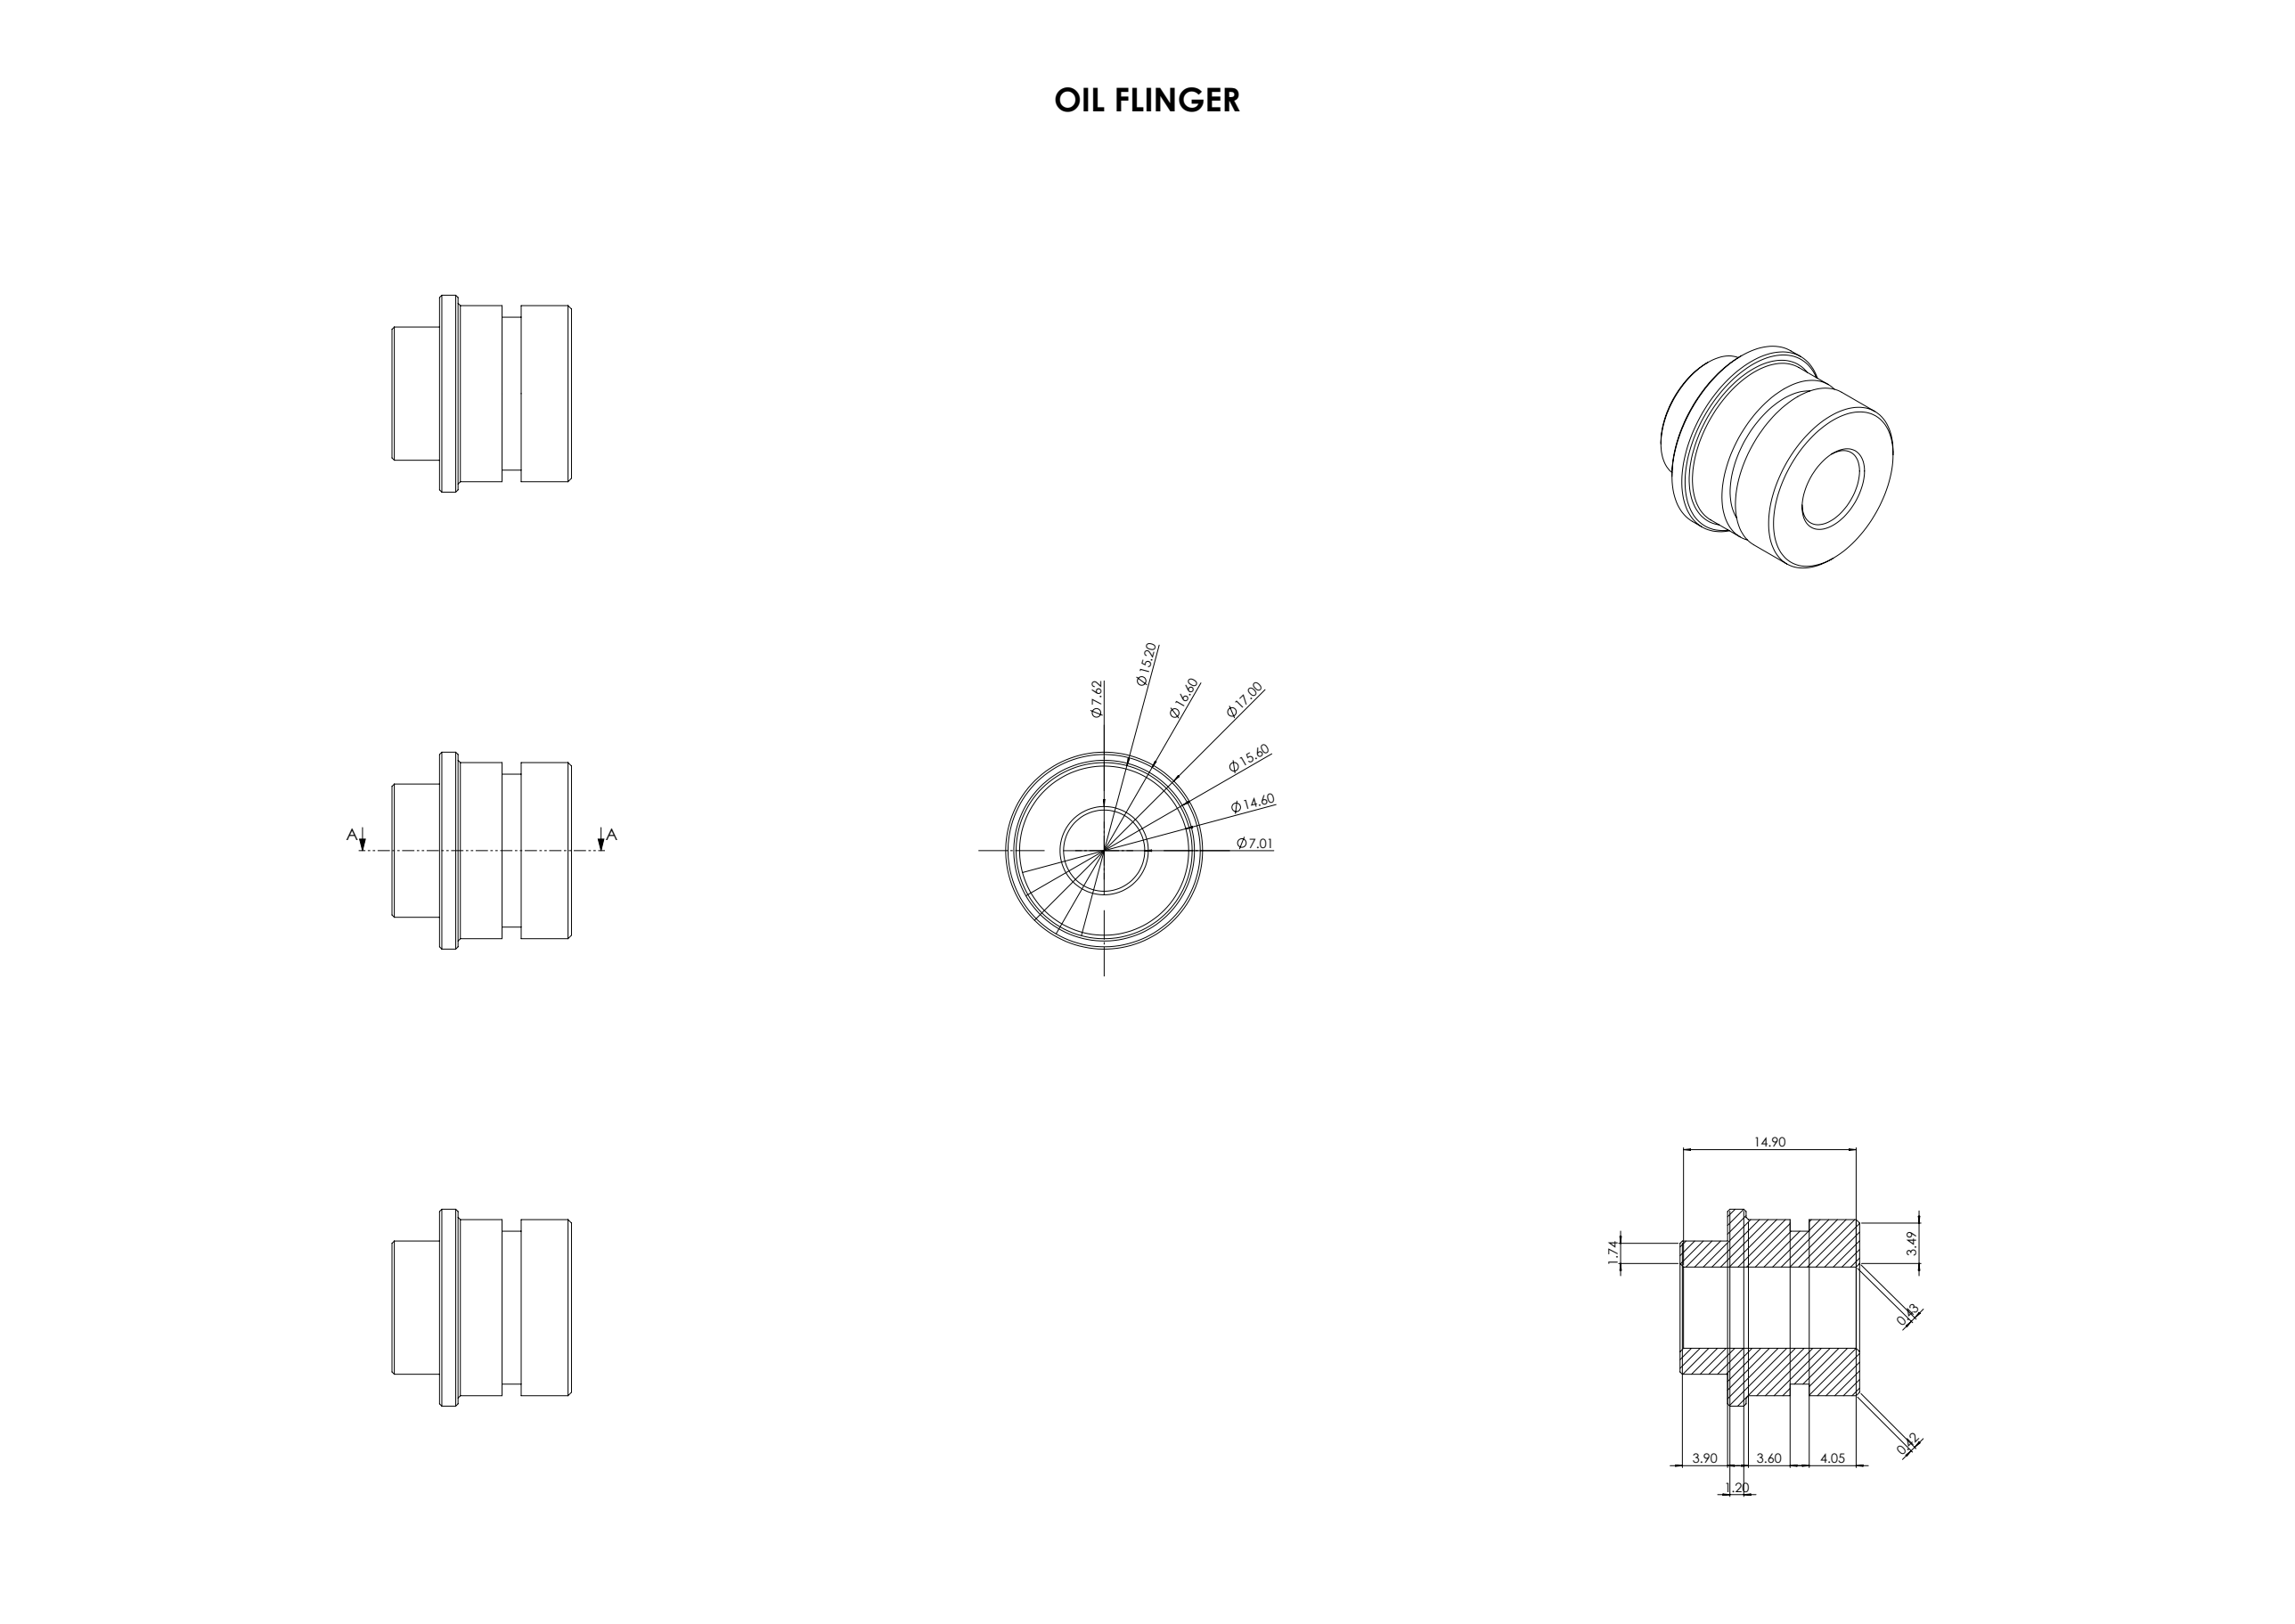
ISO-10303-21;
HEADER;
/* Generated by software containing ST-Developer
 * from STEP Tools, Inc. (www.steptools.com) 
 */

FILE_DESCRIPTION(
/* description */ (''),
/* implementation_level */ '2;1');

FILE_NAME(
/* name */ '07_Oil_Flinger.step',
/* time_stamp */ '2026-10-25T01:10:36-07:00',
/* author */ (''),
/* organization */ (''),
/* preprocessor_version */ 'ST-DEVELOPER v20.2',
/* originating_system */ 'Autodesk Translation Framework v15.15.0.0',
/* authorisation */ '');

FILE_SCHEMA (('AUTOMOTIVE_DESIGN { 1 0 10303 214 3 1 1 }'));
ENDSEC;

DATA;
#10=MECHANICAL_DESIGN_GEOMETRIC_PRESENTATION_REPRESENTATION('',(#1299),#60365);
#71=SHAPE_REPRESENTATION_RELATIONSHIP('SRR','None',#60411,#81);
#81=ADVANCED_BREP_SHAPE_REPRESENTATION('',(#91),#60359);
#91=MANIFOLD_SOLID_BREP('Body1',#18301);
#229=FACE_BOUND('',#2864,.T.);
#230=FACE_BOUND('',#2866,.T.);
#231=FACE_BOUND('',#2871,.T.);
#232=FACE_BOUND('',#2872,.T.);
#233=FACE_BOUND('',#2873,.T.);
#234=FACE_BOUND('',#2874,.T.);
#235=FACE_BOUND('',#2875,.T.);
#236=FACE_BOUND('',#2876,.T.);
#237=FACE_BOUND('',#2877,.T.);
#238=FACE_BOUND('',#2882,.T.);
#239=FACE_BOUND('',#2887,.T.);
#240=FACE_BOUND('',#2892,.T.);
#592=PLANE('',#19167);
#593=PLANE('',#19171);
#594=PLANE('',#19175);
#595=PLANE('',#19179);
#596=PLANE('',#19183);
#597=PLANE('',#19187);
#598=PLANE('',#19191);
#599=PLANE('',#19193);
#600=PLANE('',#19202);
#601=PLANE('',#19210);
#602=PLANE('',#19217);
#603=PLANE('',#19225);
#915=CONICAL_SURFACE('',#19197,5.65,0.785398163397449);
#916=CONICAL_SURFACE('',#19204,8.4,0.785398163397446);
#917=CONICAL_SURFACE('',#19208,8.4,0.785398163397446);
#918=CONICAL_SURFACE('',#19212,7.7,0.785398163397448);
#919=CONICAL_SURFACE('',#19215,7.45,0.785398163397448);
#920=CONICAL_SURFACE('',#19219,3.6575,0.7936624380571);
#921=CONICAL_SURFACE('',#19223,3.6575,0.7936624380571);
#1299=STYLED_ITEM('',(#60520),#91);
#1854=FACE_OUTER_BOUND('',#2850,.T.);
#1855=FACE_OUTER_BOUND('',#2851,.T.);
#1856=FACE_OUTER_BOUND('',#2852,.T.);
#1857=FACE_OUTER_BOUND('',#2853,.T.);
#1858=FACE_OUTER_BOUND('',#2854,.T.);
#1859=FACE_OUTER_BOUND('',#2855,.T.);
#1860=FACE_OUTER_BOUND('',#2856,.T.);
#1861=FACE_OUTER_BOUND('',#2857,.T.);
#1862=FACE_OUTER_BOUND('',#2858,.T.);
#1863=FACE_OUTER_BOUND('',#2859,.T.);
#1864=FACE_OUTER_BOUND('',#2860,.T.);
#1865=FACE_OUTER_BOUND('',#2861,.T.);
#1866=FACE_OUTER_BOUND('',#2862,.T.);
#1867=FACE_OUTER_BOUND('',#2863,.T.);
#1868=FACE_OUTER_BOUND('',#2865,.T.);
#1869=FACE_OUTER_BOUND('',#2867,.T.);
#1870=FACE_OUTER_BOUND('',#2868,.T.);
#1871=FACE_OUTER_BOUND('',#2869,.T.);
#1872=FACE_OUTER_BOUND('',#2870,.T.);
#1873=FACE_OUTER_BOUND('',#2878,.T.);
#1874=FACE_OUTER_BOUND('',#2879,.T.);
#1875=FACE_OUTER_BOUND('',#2880,.T.);
#1876=FACE_OUTER_BOUND('',#2881,.T.);
#1877=FACE_OUTER_BOUND('',#2883,.T.);
#1878=FACE_OUTER_BOUND('',#2884,.T.);
#1879=FACE_OUTER_BOUND('',#2885,.T.);
#1880=FACE_OUTER_BOUND('',#2886,.T.);
#1881=FACE_OUTER_BOUND('',#2888,.T.);
#1882=FACE_OUTER_BOUND('',#2889,.T.);
#1883=FACE_OUTER_BOUND('',#2890,.T.);
#1884=FACE_OUTER_BOUND('',#2891,.T.);
#2850=EDGE_LOOP('',(#14883,#14884,#14885,#14886));
#2851=EDGE_LOOP('',(#14887));
#2852=EDGE_LOOP('',(#14888,#14889,#14890,#14891));
#2853=EDGE_LOOP('',(#14892));
#2854=EDGE_LOOP('',(#14893,#14894,#14895,#14896));
#2855=EDGE_LOOP('',(#14897));
#2856=EDGE_LOOP('',(#14898,#14899,#14900,#14901));
#2857=EDGE_LOOP('',(#14902));
#2858=EDGE_LOOP('',(#14903,#14904,#14905,#14906));
#2859=EDGE_LOOP('',(#14907));
#2860=EDGE_LOOP('',(#14908,#14909,#14910,#14911));
#2861=EDGE_LOOP('',(#14912));
#2862=EDGE_LOOP('',(#14913,#14914,#14915,#14916));
#2863=EDGE_LOOP('',(#14917));
#2864=EDGE_LOOP('',(#14918));
#2865=EDGE_LOOP('',(#14919));
#2866=EDGE_LOOP('',(#14920));
#2867=EDGE_LOOP('',(#14921,#14922,#14923,#14924));
#2868=EDGE_LOOP('',(#14925,#14926,#14927,#14928));
#2869=EDGE_LOOP('',(#14929,#14930,#14931,#14932));
#2870=EDGE_LOOP('',(#14933));
#2871=EDGE_LOOP('',(#14934));
#2872=EDGE_LOOP('',(#14935));
#2873=EDGE_LOOP('',(#14936));
#2874=EDGE_LOOP('',(#14937));
#2875=EDGE_LOOP('',(#14938));
#2876=EDGE_LOOP('',(#14939));
#2877=EDGE_LOOP('',(#14940));
#2878=EDGE_LOOP('',(#14941,#14942,#14943,#14944));
#2879=EDGE_LOOP('',(#14945,#14946,#14947,#14948));
#2880=EDGE_LOOP('',(#14949,#14950,#14951,#14952));
#2881=EDGE_LOOP('',(#14953));
#2882=EDGE_LOOP('',(#14954));
#2883=EDGE_LOOP('',(#14955,#14956,#14957,#14958));
#2884=EDGE_LOOP('',(#14959,#14960,#14961,#14962));
#2885=EDGE_LOOP('',(#14963,#14964,#14965,#14966));
#2886=EDGE_LOOP('',(#14967));
#2887=EDGE_LOOP('',(#14968));
#2888=EDGE_LOOP('',(#14969,#14970,#14971,#14972));
#2889=EDGE_LOOP('',(#14973,#14974,#14975,#14976));
#2890=EDGE_LOOP('',(#14977,#14978,#14979,#14980));
#2891=EDGE_LOOP('',(#14981));
#2892=EDGE_LOOP('',(#14982));
#3537=CIRCLE('',#19165,0.600000000000001);
#3538=CIRCLE('',#19166,0.600000000000001);
#3539=CIRCLE('',#19169,0.6);
#3540=CIRCLE('',#19170,0.6);
#3541=CIRCLE('',#19173,0.600000000000001);
#3542=CIRCLE('',#19174,0.600000000000001);
#3543=CIRCLE('',#19177,0.600000000000001);
#3544=CIRCLE('',#19178,0.600000000000001);
#3545=CIRCLE('',#19181,0.6);
#3546=CIRCLE('',#19182,0.6);
#3547=CIRCLE('',#19185,0.600000000000001);
#3548=CIRCLE('',#19186,0.600000000000001);
#3549=CIRCLE('',#19189,6.6);
#3550=CIRCLE('',#19190,6.6);
#3551=CIRCLE('',#19192,7.6);
#3552=CIRCLE('',#19194,7.6);
#3553=CIRCLE('',#19196,7.6);
#3554=CIRCLE('',#19198,5.75);
#3555=CIRCLE('',#19199,5.55);
#3556=CIRCLE('',#19201,5.75);
#3557=CIRCLE('',#19203,8.3);
#3558=CIRCLE('',#19205,8.5);
#3559=CIRCLE('',#19207,8.5);
#3560=CIRCLE('',#19209,8.3);
#3561=CIRCLE('',#19211,7.8);
#3562=CIRCLE('',#19213,7.6);
#3563=CIRCLE('',#19216,7.3);
#3564=CIRCLE('',#19218,3.81);
#3565=CIRCLE('',#19220,3.505);
#3566=CIRCLE('',#19222,3.505);
#3567=CIRCLE('',#19224,3.81);
#5321=LINE('',#44964,#6733);
#5322=LINE('',#44971,#6734);
#5323=LINE('',#44978,#6735);
#5324=LINE('',#44985,#6736);
#5325=LINE('',#44992,#6737);
#5326=LINE('',#44999,#6738);
#5327=LINE('',#45006,#6739);
#5328=LINE('',#45017,#6740);
#5329=LINE('',#45022,#6741);
#5330=LINE('',#45027,#6742);
#5331=LINE('',#45034,#6743);
#5332=LINE('',#45038,#6744);
#5333=LINE('',#45042,#6745);
#5334=LINE('',#45049,#6746);
#5335=LINE('',#45051,#6747);
#5336=LINE('',#45055,#6748);
#5337=LINE('',#45061,#6749);
#5338=LINE('',#45065,#6750);
#5339=LINE('',#45069,#6751);
#6733=VECTOR('',#21995,0.600000000000001);
#6734=VECTOR('',#22004,0.6);
#6735=VECTOR('',#22013,0.600000000000001);
#6736=VECTOR('',#22022,0.600000000000001);
#6737=VECTOR('',#22031,0.6);
#6738=VECTOR('',#22040,0.600000000000001);
#6739=VECTOR('',#22049,6.6);
#6740=VECTOR('',#22064,7.6);
#6741=VECTOR('',#22069,5.65);
#6742=VECTOR('',#22076,5.75);
#6743=VECTOR('',#22085,8.4);
#6744=VECTOR('',#22090,8.5);
#6745=VECTOR('',#22095,8.4);
#6746=VECTOR('',#22104,7.7);
#6747=VECTOR('',#22107,7.6);
#6748=VECTOR('',#22112,7.45);
#6749=VECTOR('',#22119,3.6575);
#6750=VECTOR('',#22124,3.505);
#6751=VECTOR('',#22129,3.6575);
#8337=VERTEX_POINT('',#44961);
#8338=VERTEX_POINT('',#44963);
#8339=VERTEX_POINT('',#44968);
#8340=VERTEX_POINT('',#44970);
#8341=VERTEX_POINT('',#44975);
#8342=VERTEX_POINT('',#44977);
#8343=VERTEX_POINT('',#44982);
#8344=VERTEX_POINT('',#44984);
#8345=VERTEX_POINT('',#44989);
#8346=VERTEX_POINT('',#44991);
#8347=VERTEX_POINT('',#44996);
#8348=VERTEX_POINT('',#44998);
#8349=VERTEX_POINT('',#45003);
#8350=VERTEX_POINT('',#45005);
#8351=VERTEX_POINT('',#45009);
#8352=VERTEX_POINT('',#45012);
#8353=VERTEX_POINT('',#45015);
#8354=VERTEX_POINT('',#45019);
#8355=VERTEX_POINT('',#45021);
#8356=VERTEX_POINT('',#45025);
#8357=VERTEX_POINT('',#45029);
#8358=VERTEX_POINT('',#45032);
#8359=VERTEX_POINT('',#45036);
#8360=VERTEX_POINT('',#45040);
#8361=VERTEX_POINT('',#45044);
#8362=VERTEX_POINT('',#45047);
#8363=VERTEX_POINT('',#45053);
#8364=VERTEX_POINT('',#45057);
#8365=VERTEX_POINT('',#45060);
#8366=VERTEX_POINT('',#45064);
#8367=VERTEX_POINT('',#45068);
#10649=EDGE_CURVE('',#8337,#8337,#3537,.T.);
#10650=EDGE_CURVE('',#8337,#8338,#5321,.T.);
#10651=EDGE_CURVE('',#8338,#8338,#3538,.T.);
#10652=EDGE_CURVE('',#8339,#8339,#3539,.T.);
#10653=EDGE_CURVE('',#8339,#8340,#5322,.T.);
#10654=EDGE_CURVE('',#8340,#8340,#3540,.T.);
#10655=EDGE_CURVE('',#8341,#8341,#3541,.T.);
#10656=EDGE_CURVE('',#8341,#8342,#5323,.T.);
#10657=EDGE_CURVE('',#8342,#8342,#3542,.T.);
#10658=EDGE_CURVE('',#8343,#8343,#3543,.T.);
#10659=EDGE_CURVE('',#8343,#8344,#5324,.T.);
#10660=EDGE_CURVE('',#8344,#8344,#3544,.T.);
#10661=EDGE_CURVE('',#8345,#8345,#3545,.T.);
#10662=EDGE_CURVE('',#8345,#8346,#5325,.T.);
#10663=EDGE_CURVE('',#8346,#8346,#3546,.T.);
#10664=EDGE_CURVE('',#8347,#8347,#3547,.T.);
#10665=EDGE_CURVE('',#8347,#8348,#5326,.T.);
#10666=EDGE_CURVE('',#8348,#8348,#3548,.T.);
#10667=EDGE_CURVE('',#8349,#8349,#3549,.T.);
#10668=EDGE_CURVE('',#8349,#8350,#5327,.T.);
#10669=EDGE_CURVE('',#8350,#8350,#3550,.T.);
#10670=EDGE_CURVE('',#8351,#8351,#3551,.T.);
#10671=EDGE_CURVE('',#8352,#8352,#3552,.T.);
#10672=EDGE_CURVE('',#8353,#8353,#3553,.T.);
#10673=EDGE_CURVE('',#8353,#8352,#5328,.T.);
#10674=EDGE_CURVE('',#8354,#8354,#3554,.T.);
#10675=EDGE_CURVE('',#8354,#8355,#5329,.T.);
#10676=EDGE_CURVE('',#8355,#8355,#3555,.T.);
#10677=EDGE_CURVE('',#8356,#8356,#3556,.T.);
#10678=EDGE_CURVE('',#8356,#8354,#5330,.T.);
#10679=EDGE_CURVE('',#8357,#8357,#3557,.T.);
#10680=EDGE_CURVE('',#8358,#8358,#3558,.T.);
#10681=EDGE_CURVE('',#8358,#8357,#5331,.T.);
#10682=EDGE_CURVE('',#8359,#8359,#3559,.T.);
#10683=EDGE_CURVE('',#8359,#8358,#5332,.T.);
#10684=EDGE_CURVE('',#8360,#8360,#3560,.T.);
#10685=EDGE_CURVE('',#8360,#8359,#5333,.T.);
#10686=EDGE_CURVE('',#8361,#8361,#3561,.T.);
#10687=EDGE_CURVE('',#8362,#8362,#3562,.T.);
#10688=EDGE_CURVE('',#8362,#8361,#5334,.T.);
#10689=EDGE_CURVE('',#8351,#8362,#5335,.T.);
#10690=EDGE_CURVE('',#8363,#8363,#3563,.T.);
#10691=EDGE_CURVE('',#8363,#8353,#5336,.T.);
#10692=EDGE_CURVE('',#8364,#8364,#3564,.T.);
#10693=EDGE_CURVE('',#8364,#8365,#5337,.T.);
#10694=EDGE_CURVE('',#8365,#8365,#3565,.T.);
#10695=EDGE_CURVE('',#8365,#8366,#5338,.T.);
#10696=EDGE_CURVE('',#8366,#8366,#3566,.T.);
#10697=EDGE_CURVE('',#8366,#8367,#5339,.T.);
#10698=EDGE_CURVE('',#8367,#8367,#3567,.T.);
#14883=ORIENTED_EDGE('',*,*,#10649,.F.);
#14884=ORIENTED_EDGE('',*,*,#10650,.T.);
#14885=ORIENTED_EDGE('',*,*,#10651,.T.);
#14886=ORIENTED_EDGE('',*,*,#10650,.F.);
#14887=ORIENTED_EDGE('',*,*,#10651,.F.);
#14888=ORIENTED_EDGE('',*,*,#10652,.F.);
#14889=ORIENTED_EDGE('',*,*,#10653,.T.);
#14890=ORIENTED_EDGE('',*,*,#10654,.T.);
#14891=ORIENTED_EDGE('',*,*,#10653,.F.);
#14892=ORIENTED_EDGE('',*,*,#10654,.F.);
#14893=ORIENTED_EDGE('',*,*,#10655,.F.);
#14894=ORIENTED_EDGE('',*,*,#10656,.T.);
#14895=ORIENTED_EDGE('',*,*,#10657,.T.);
#14896=ORIENTED_EDGE('',*,*,#10656,.F.);
#14897=ORIENTED_EDGE('',*,*,#10657,.F.);
#14898=ORIENTED_EDGE('',*,*,#10658,.F.);
#14899=ORIENTED_EDGE('',*,*,#10659,.T.);
#14900=ORIENTED_EDGE('',*,*,#10660,.T.);
#14901=ORIENTED_EDGE('',*,*,#10659,.F.);
#14902=ORIENTED_EDGE('',*,*,#10660,.F.);
#14903=ORIENTED_EDGE('',*,*,#10661,.F.);
#14904=ORIENTED_EDGE('',*,*,#10662,.T.);
#14905=ORIENTED_EDGE('',*,*,#10663,.T.);
#14906=ORIENTED_EDGE('',*,*,#10662,.F.);
#14907=ORIENTED_EDGE('',*,*,#10663,.F.);
#14908=ORIENTED_EDGE('',*,*,#10664,.F.);
#14909=ORIENTED_EDGE('',*,*,#10665,.T.);
#14910=ORIENTED_EDGE('',*,*,#10666,.T.);
#14911=ORIENTED_EDGE('',*,*,#10665,.F.);
#14912=ORIENTED_EDGE('',*,*,#10666,.F.);
#14913=ORIENTED_EDGE('',*,*,#10667,.T.);
#14914=ORIENTED_EDGE('',*,*,#10668,.T.);
#14915=ORIENTED_EDGE('',*,*,#10669,.F.);
#14916=ORIENTED_EDGE('',*,*,#10668,.F.);
#14917=ORIENTED_EDGE('',*,*,#10670,.F.);
#14918=ORIENTED_EDGE('',*,*,#10667,.F.);
#14919=ORIENTED_EDGE('',*,*,#10671,.F.);
#14920=ORIENTED_EDGE('',*,*,#10669,.T.);
#14921=ORIENTED_EDGE('',*,*,#10672,.F.);
#14922=ORIENTED_EDGE('',*,*,#10673,.T.);
#14923=ORIENTED_EDGE('',*,*,#10671,.T.);
#14924=ORIENTED_EDGE('',*,*,#10673,.F.);
#14925=ORIENTED_EDGE('',*,*,#10674,.F.);
#14926=ORIENTED_EDGE('',*,*,#10675,.T.);
#14927=ORIENTED_EDGE('',*,*,#10676,.T.);
#14928=ORIENTED_EDGE('',*,*,#10675,.F.);
#14929=ORIENTED_EDGE('',*,*,#10677,.F.);
#14930=ORIENTED_EDGE('',*,*,#10678,.T.);
#14931=ORIENTED_EDGE('',*,*,#10674,.T.);
#14932=ORIENTED_EDGE('',*,*,#10678,.F.);
#14933=ORIENTED_EDGE('',*,*,#10679,.F.);
#14934=ORIENTED_EDGE('',*,*,#10677,.T.);
#14935=ORIENTED_EDGE('',*,*,#10664,.T.);
#14936=ORIENTED_EDGE('',*,*,#10661,.T.);
#14937=ORIENTED_EDGE('',*,*,#10658,.T.);
#14938=ORIENTED_EDGE('',*,*,#10655,.T.);
#14939=ORIENTED_EDGE('',*,*,#10652,.T.);
#14940=ORIENTED_EDGE('',*,*,#10649,.T.);
#14941=ORIENTED_EDGE('',*,*,#10680,.F.);
#14942=ORIENTED_EDGE('',*,*,#10681,.T.);
#14943=ORIENTED_EDGE('',*,*,#10679,.T.);
#14944=ORIENTED_EDGE('',*,*,#10681,.F.);
#14945=ORIENTED_EDGE('',*,*,#10682,.F.);
#14946=ORIENTED_EDGE('',*,*,#10683,.T.);
#14947=ORIENTED_EDGE('',*,*,#10680,.T.);
#14948=ORIENTED_EDGE('',*,*,#10683,.F.);
#14949=ORIENTED_EDGE('',*,*,#10684,.F.);
#14950=ORIENTED_EDGE('',*,*,#10685,.T.);
#14951=ORIENTED_EDGE('',*,*,#10682,.T.);
#14952=ORIENTED_EDGE('',*,*,#10685,.F.);
#14953=ORIENTED_EDGE('',*,*,#10684,.T.);
#14954=ORIENTED_EDGE('',*,*,#10686,.F.);
#14955=ORIENTED_EDGE('',*,*,#10687,.F.);
#14956=ORIENTED_EDGE('',*,*,#10688,.T.);
#14957=ORIENTED_EDGE('',*,*,#10686,.T.);
#14958=ORIENTED_EDGE('',*,*,#10688,.F.);
#14959=ORIENTED_EDGE('',*,*,#10670,.T.);
#14960=ORIENTED_EDGE('',*,*,#10689,.T.);
#14961=ORIENTED_EDGE('',*,*,#10687,.T.);
#14962=ORIENTED_EDGE('',*,*,#10689,.F.);
#14963=ORIENTED_EDGE('',*,*,#10690,.F.);
#14964=ORIENTED_EDGE('',*,*,#10691,.T.);
#14965=ORIENTED_EDGE('',*,*,#10672,.T.);
#14966=ORIENTED_EDGE('',*,*,#10691,.F.);
#14967=ORIENTED_EDGE('',*,*,#10690,.T.);
#14968=ORIENTED_EDGE('',*,*,#10692,.F.);
#14969=ORIENTED_EDGE('',*,*,#10692,.T.);
#14970=ORIENTED_EDGE('',*,*,#10693,.T.);
#14971=ORIENTED_EDGE('',*,*,#10694,.F.);
#14972=ORIENTED_EDGE('',*,*,#10693,.F.);
#14973=ORIENTED_EDGE('',*,*,#10694,.T.);
#14974=ORIENTED_EDGE('',*,*,#10695,.T.);
#14975=ORIENTED_EDGE('',*,*,#10696,.F.);
#14976=ORIENTED_EDGE('',*,*,#10695,.F.);
#14977=ORIENTED_EDGE('',*,*,#10696,.T.);
#14978=ORIENTED_EDGE('',*,*,#10697,.T.);
#14979=ORIENTED_EDGE('',*,*,#10698,.F.);
#14980=ORIENTED_EDGE('',*,*,#10697,.F.);
#14981=ORIENTED_EDGE('',*,*,#10676,.F.);
#14982=ORIENTED_EDGE('',*,*,#10698,.T.);
#17302=CYLINDRICAL_SURFACE('',#19164,0.600000000000001);
#17303=CYLINDRICAL_SURFACE('',#19168,0.6);
#17304=CYLINDRICAL_SURFACE('',#19172,0.600000000000001);
#17305=CYLINDRICAL_SURFACE('',#19176,0.600000000000001);
#17306=CYLINDRICAL_SURFACE('',#19180,0.6);
#17307=CYLINDRICAL_SURFACE('',#19184,0.600000000000001);
#17308=CYLINDRICAL_SURFACE('',#19188,6.6);
#17309=CYLINDRICAL_SURFACE('',#19195,7.6);
#17310=CYLINDRICAL_SURFACE('',#19200,5.75);
#17311=CYLINDRICAL_SURFACE('',#19206,8.5);
#17312=CYLINDRICAL_SURFACE('',#19214,7.6);
#17313=CYLINDRICAL_SURFACE('',#19221,3.505);
#17882=ADVANCED_FACE('',(#1854),#17302,.F.);
#17883=ADVANCED_FACE('',(#1855),#592,.F.);
#17884=ADVANCED_FACE('',(#1856),#17303,.F.);
#17885=ADVANCED_FACE('',(#1857),#593,.F.);
#17886=ADVANCED_FACE('',(#1858),#17304,.F.);
#17887=ADVANCED_FACE('',(#1859),#594,.F.);
#17888=ADVANCED_FACE('',(#1860),#17305,.F.);
#17889=ADVANCED_FACE('',(#1861),#595,.F.);
#17890=ADVANCED_FACE('',(#1862),#17306,.F.);
#17891=ADVANCED_FACE('',(#1863),#596,.F.);
#17892=ADVANCED_FACE('',(#1864),#17307,.F.);
#17893=ADVANCED_FACE('',(#1865),#597,.F.);
#17894=ADVANCED_FACE('',(#1866),#17308,.T.);
#17895=ADVANCED_FACE('',(#1867,#229),#598,.F.);
#17896=ADVANCED_FACE('',(#1868,#230),#599,.F.);
#17897=ADVANCED_FACE('',(#1869),#17309,.T.);
#17898=ADVANCED_FACE('',(#1870),#915,.T.);
#17899=ADVANCED_FACE('',(#1871),#17310,.T.);
#17900=ADVANCED_FACE('',(#1872,#231,#232,#233,#234,#235,#236,#237),#600,
 .T.);
#17901=ADVANCED_FACE('',(#1873),#916,.T.);
#17902=ADVANCED_FACE('',(#1874),#17311,.T.);
#17903=ADVANCED_FACE('',(#1875),#917,.T.);
#17904=ADVANCED_FACE('',(#1876,#238),#601,.T.);
#17905=ADVANCED_FACE('',(#1877),#918,.T.);
#17906=ADVANCED_FACE('',(#1878),#17312,.T.);
#17907=ADVANCED_FACE('',(#1879),#919,.T.);
#17908=ADVANCED_FACE('',(#1880,#239),#602,.T.);
#17909=ADVANCED_FACE('',(#1881),#920,.F.);
#17910=ADVANCED_FACE('',(#1882),#17313,.F.);
#17911=ADVANCED_FACE('',(#1883),#921,.F.);
#17912=ADVANCED_FACE('',(#1884,#240),#603,.T.);
#18301=CLOSED_SHELL('',(#17882,#17883,#17884,#17885,#17886,#17887,#17888,
#17889,#17890,#17891,#17892,#17893,#17894,#17895,#17896,#17897,#17898,#17899,
#17900,#17901,#17902,#17903,#17904,#17905,#17906,#17907,#17908,#17909,#17910,
#17911,#17912));
#19163=AXIS2_PLACEMENT_3D('',#44959,#21989,#21990);
#19164=AXIS2_PLACEMENT_3D('',#44960,#21991,#21992);
#19165=AXIS2_PLACEMENT_3D('',#44962,#21993,#21994);
#19166=AXIS2_PLACEMENT_3D('',#44965,#21996,#21997);
#19167=AXIS2_PLACEMENT_3D('',#44966,#21998,#21999);
#19168=AXIS2_PLACEMENT_3D('',#44967,#22000,#22001);
#19169=AXIS2_PLACEMENT_3D('',#44969,#22002,#22003);
#19170=AXIS2_PLACEMENT_3D('',#44972,#22005,#22006);
#19171=AXIS2_PLACEMENT_3D('',#44973,#22007,#22008);
#19172=AXIS2_PLACEMENT_3D('',#44974,#22009,#22010);
#19173=AXIS2_PLACEMENT_3D('',#44976,#22011,#22012);
#19174=AXIS2_PLACEMENT_3D('',#44979,#22014,#22015);
#19175=AXIS2_PLACEMENT_3D('',#44980,#22016,#22017);
#19176=AXIS2_PLACEMENT_3D('',#44981,#22018,#22019);
#19177=AXIS2_PLACEMENT_3D('',#44983,#22020,#22021);
#19178=AXIS2_PLACEMENT_3D('',#44986,#22023,#22024);
#19179=AXIS2_PLACEMENT_3D('',#44987,#22025,#22026);
#19180=AXIS2_PLACEMENT_3D('',#44988,#22027,#22028);
#19181=AXIS2_PLACEMENT_3D('',#44990,#22029,#22030);
#19182=AXIS2_PLACEMENT_3D('',#44993,#22032,#22033);
#19183=AXIS2_PLACEMENT_3D('',#44994,#22034,#22035);
#19184=AXIS2_PLACEMENT_3D('',#44995,#22036,#22037);
#19185=AXIS2_PLACEMENT_3D('',#44997,#22038,#22039);
#19186=AXIS2_PLACEMENT_3D('',#45000,#22041,#22042);
#19187=AXIS2_PLACEMENT_3D('',#45001,#22043,#22044);
#19188=AXIS2_PLACEMENT_3D('',#45002,#22045,#22046);
#19189=AXIS2_PLACEMENT_3D('',#45004,#22047,#22048);
#19190=AXIS2_PLACEMENT_3D('',#45007,#22050,#22051);
#19191=AXIS2_PLACEMENT_3D('',#45008,#22052,#22053);
#19192=AXIS2_PLACEMENT_3D('',#45010,#22054,#22055);
#19193=AXIS2_PLACEMENT_3D('',#45011,#22056,#22057);
#19194=AXIS2_PLACEMENT_3D('',#45013,#22058,#22059);
#19195=AXIS2_PLACEMENT_3D('',#45014,#22060,#22061);
#19196=AXIS2_PLACEMENT_3D('',#45016,#22062,#22063);
#19197=AXIS2_PLACEMENT_3D('',#45018,#22065,#22066);
#19198=AXIS2_PLACEMENT_3D('',#45020,#22067,#22068);
#19199=AXIS2_PLACEMENT_3D('',#45023,#22070,#22071);
#19200=AXIS2_PLACEMENT_3D('',#45024,#22072,#22073);
#19201=AXIS2_PLACEMENT_3D('',#45026,#22074,#22075);
#19202=AXIS2_PLACEMENT_3D('',#45028,#22077,#22078);
#19203=AXIS2_PLACEMENT_3D('',#45030,#22079,#22080);
#19204=AXIS2_PLACEMENT_3D('',#45031,#22081,#22082);
#19205=AXIS2_PLACEMENT_3D('',#45033,#22083,#22084);
#19206=AXIS2_PLACEMENT_3D('',#45035,#22086,#22087);
#19207=AXIS2_PLACEMENT_3D('',#45037,#22088,#22089);
#19208=AXIS2_PLACEMENT_3D('',#45039,#22091,#22092);
#19209=AXIS2_PLACEMENT_3D('',#45041,#22093,#22094);
#19210=AXIS2_PLACEMENT_3D('',#45043,#22096,#22097);
#19211=AXIS2_PLACEMENT_3D('',#45045,#22098,#22099);
#19212=AXIS2_PLACEMENT_3D('',#45046,#22100,#22101);
#19213=AXIS2_PLACEMENT_3D('',#45048,#22102,#22103);
#19214=AXIS2_PLACEMENT_3D('',#45050,#22105,#22106);
#19215=AXIS2_PLACEMENT_3D('',#45052,#22108,#22109);
#19216=AXIS2_PLACEMENT_3D('',#45054,#22110,#22111);
#19217=AXIS2_PLACEMENT_3D('',#45056,#22113,#22114);
#19218=AXIS2_PLACEMENT_3D('',#45058,#22115,#22116);
#19219=AXIS2_PLACEMENT_3D('',#45059,#22117,#22118);
#19220=AXIS2_PLACEMENT_3D('',#45062,#22120,#22121);
#19221=AXIS2_PLACEMENT_3D('',#45063,#22122,#22123);
#19222=AXIS2_PLACEMENT_3D('',#45066,#22125,#22126);
#19223=AXIS2_PLACEMENT_3D('',#45067,#22127,#22128);
#19224=AXIS2_PLACEMENT_3D('',#45070,#22130,#22131);
#19225=AXIS2_PLACEMENT_3D('',#45071,#22132,#22133);
#21989=DIRECTION('axis',(0.,0.,1.));
#21990=DIRECTION('refdir',(1.,0.,0.));
#21991=DIRECTION('center_axis',(1.,0.,0.));
#21992=DIRECTION('ref_axis',(0.,0.,-1.));
#21993=DIRECTION('center_axis',(1.,0.,0.));
#21994=DIRECTION('ref_axis',(0.,0.,-1.));
#21995=DIRECTION('',(1.,0.,0.));
#21996=DIRECTION('center_axis',(1.,0.,0.));
#21997=DIRECTION('ref_axis',(0.,0.,-1.));
#21998=DIRECTION('center_axis',(1.,0.,0.));
#21999=DIRECTION('ref_axis',(0.,0.,-1.));
#22000=DIRECTION('center_axis',(1.,0.,0.));
#22001=DIRECTION('ref_axis',(0.,0.,-1.));
#22002=DIRECTION('center_axis',(1.,0.,0.));
#22003=DIRECTION('ref_axis',(0.,0.,-1.));
#22004=DIRECTION('',(1.,0.,0.));
#22005=DIRECTION('center_axis',(1.,0.,0.));
#22006=DIRECTION('ref_axis',(0.,0.,-1.));
#22007=DIRECTION('center_axis',(1.,0.,0.));
#22008=DIRECTION('ref_axis',(0.,0.,-1.));
#22009=DIRECTION('center_axis',(1.,0.,0.));
#22010=DIRECTION('ref_axis',(0.,0.,-1.));
#22011=DIRECTION('center_axis',(1.,0.,0.));
#22012=DIRECTION('ref_axis',(0.,0.,-1.));
#22013=DIRECTION('',(1.,0.,0.));
#22014=DIRECTION('center_axis',(1.,0.,0.));
#22015=DIRECTION('ref_axis',(0.,0.,-1.));
#22016=DIRECTION('center_axis',(1.,0.,0.));
#22017=DIRECTION('ref_axis',(0.,0.,-1.));
#22018=DIRECTION('center_axis',(1.,0.,0.));
#22019=DIRECTION('ref_axis',(0.,0.,-1.));
#22020=DIRECTION('center_axis',(1.,0.,0.));
#22021=DIRECTION('ref_axis',(0.,0.,-1.));
#22022=DIRECTION('',(1.,0.,0.));
#22023=DIRECTION('center_axis',(1.,0.,0.));
#22024=DIRECTION('ref_axis',(0.,0.,-1.));
#22025=DIRECTION('center_axis',(1.,0.,0.));
#22026=DIRECTION('ref_axis',(0.,0.,-1.));
#22027=DIRECTION('center_axis',(1.,0.,0.));
#22028=DIRECTION('ref_axis',(0.,0.,-1.));
#22029=DIRECTION('center_axis',(1.,0.,0.));
#22030=DIRECTION('ref_axis',(0.,0.,-1.));
#22031=DIRECTION('',(1.,0.,0.));
#22032=DIRECTION('center_axis',(1.,0.,0.));
#22033=DIRECTION('ref_axis',(0.,0.,-1.));
#22034=DIRECTION('center_axis',(1.,0.,0.));
#22035=DIRECTION('ref_axis',(0.,0.,-1.));
#22036=DIRECTION('center_axis',(1.,0.,0.));
#22037=DIRECTION('ref_axis',(0.,0.,-1.));
#22038=DIRECTION('center_axis',(1.,0.,0.));
#22039=DIRECTION('ref_axis',(0.,0.,-1.));
#22040=DIRECTION('',(1.,0.,0.));
#22041=DIRECTION('center_axis',(1.,0.,0.));
#22042=DIRECTION('ref_axis',(0.,0.,-1.));
#22043=DIRECTION('center_axis',(1.,0.,0.));
#22044=DIRECTION('ref_axis',(0.,0.,-1.));
#22045=DIRECTION('center_axis',(1.,0.,0.));
#22046=DIRECTION('ref_axis',(0.,1.,0.));
#22047=DIRECTION('center_axis',(1.,0.,0.));
#22048=DIRECTION('ref_axis',(0.,0.,-1.));
#22049=DIRECTION('',(1.,0.,0.));
#22050=DIRECTION('center_axis',(1.,0.,0.));
#22051=DIRECTION('ref_axis',(0.,0.,-1.));
#22052=DIRECTION('center_axis',(-1.,0.,0.));
#22053=DIRECTION('ref_axis',(0.,0.,1.));
#22054=DIRECTION('center_axis',(-1.,0.,0.));
#22055=DIRECTION('ref_axis',(0.,1.,0.));
#22056=DIRECTION('center_axis',(1.,0.,0.));
#22057=DIRECTION('ref_axis',(0.,0.,-1.));
#22058=DIRECTION('center_axis',(1.,0.,0.));
#22059=DIRECTION('ref_axis',(0.,1.,0.));
#22060=DIRECTION('center_axis',(1.,0.,0.));
#22061=DIRECTION('ref_axis',(0.,1.,0.));
#22062=DIRECTION('center_axis',(1.,0.,0.));
#22063=DIRECTION('ref_axis',(0.,0.,-1.));
#22064=DIRECTION('',(-1.,0.,0.));
#22065=DIRECTION('center_axis',(1.,0.,0.));
#22066=DIRECTION('ref_axis',(0.,1.,0.));
#22067=DIRECTION('center_axis',(1.,0.,0.));
#22068=DIRECTION('ref_axis',(0.,0.,-1.));
#22069=DIRECTION('',(-0.707106781186547,0.707106781186548,8.65956056235494E-17));
#22070=DIRECTION('center_axis',(1.,0.,0.));
#22071=DIRECTION('ref_axis',(0.,0.,-1.));
#22072=DIRECTION('center_axis',(1.,0.,0.));
#22073=DIRECTION('ref_axis',(0.,1.,0.));
#22074=DIRECTION('center_axis',(1.,0.,0.));
#22075=DIRECTION('ref_axis',(0.,0.,-1.));
#22076=DIRECTION('',(-1.,0.,0.));
#22077=DIRECTION('center_axis',(-1.,0.,0.));
#22078=DIRECTION('ref_axis',(0.,0.,1.));
#22079=DIRECTION('center_axis',(1.,0.,0.));
#22080=DIRECTION('ref_axis',(0.,0.,-1.));
#22081=DIRECTION('center_axis',(1.,0.,0.));
#22082=DIRECTION('ref_axis',(0.,1.,0.));
#22083=DIRECTION('center_axis',(1.,0.,0.));
#22084=DIRECTION('ref_axis',(0.,0.,-1.));
#22085=DIRECTION('',(-0.707106781186549,0.707106781186546,8.65956056235491E-17));
#22086=DIRECTION('center_axis',(1.,0.,0.));
#22087=DIRECTION('ref_axis',(0.,1.,0.));
#22088=DIRECTION('center_axis',(1.,0.,0.));
#22089=DIRECTION('ref_axis',(0.,0.,-1.));
#22090=DIRECTION('',(-1.,0.,0.));
#22091=DIRECTION('center_axis',(-1.,0.,0.));
#22092=DIRECTION('ref_axis',(0.,1.,0.));
#22093=DIRECTION('center_axis',(1.,0.,0.));
#22094=DIRECTION('ref_axis',(0.,0.,-1.));
#22095=DIRECTION('',(-0.707106781186549,-0.707106781186546,-8.65956056235491E-17));
#22096=DIRECTION('center_axis',(1.,0.,0.));
#22097=DIRECTION('ref_axis',(0.,0.,-1.));
#22098=DIRECTION('center_axis',(1.,0.,0.));
#22099=DIRECTION('ref_axis',(0.,0.,-1.));
#22100=DIRECTION('center_axis',(-1.,0.,0.));
#22101=DIRECTION('ref_axis',(0.,1.,0.));
#22102=DIRECTION('center_axis',(1.,0.,0.));
#22103=DIRECTION('ref_axis',(0.,0.,-1.));
#22104=DIRECTION('',(-0.707106781186547,-0.707106781186547,-8.65956056235493E-17));
#22105=DIRECTION('center_axis',(1.,0.,0.));
#22106=DIRECTION('ref_axis',(0.,1.,0.));
#22107=DIRECTION('',(-1.,0.,0.));
#22108=DIRECTION('center_axis',(-1.,0.,0.));
#22109=DIRECTION('ref_axis',(0.,1.,0.));
#22110=DIRECTION('center_axis',(1.,0.,0.));
#22111=DIRECTION('ref_axis',(0.,0.,-1.));
#22112=DIRECTION('',(-0.707106781186548,-0.707106781186548,-8.65956056235493E-17));
#22113=DIRECTION('center_axis',(1.,0.,0.));
#22114=DIRECTION('ref_axis',(0.,0.,-1.));
#22115=DIRECTION('center_axis',(1.,0.,0.));
#22116=DIRECTION('ref_axis',(0.,0.,-1.));
#22117=DIRECTION('center_axis',(1.,0.,0.));
#22118=DIRECTION('ref_axis',(0.,1.,0.));
#22119=DIRECTION('',(-0.701238976116888,0.712926292385503,8.73082901997896E-17));
#22120=DIRECTION('center_axis',(1.,0.,0.));
#22121=DIRECTION('ref_axis',(0.,0.,-1.));
#22122=DIRECTION('center_axis',(1.,0.,0.));
#22123=DIRECTION('ref_axis',(0.,1.,0.));
#22124=DIRECTION('',(-1.,0.,0.));
#22125=DIRECTION('center_axis',(1.,0.,0.));
#22126=DIRECTION('ref_axis',(0.,0.,-1.));
#22127=DIRECTION('center_axis',(-1.,0.,0.));
#22128=DIRECTION('ref_axis',(0.,1.,0.));
#22129=DIRECTION('',(-0.701238976116887,-0.712926292385503,-8.73082901997896E-17));
#22130=DIRECTION('center_axis',(1.,0.,0.));
#22131=DIRECTION('ref_axis',(0.,0.,-1.));
#22132=DIRECTION('center_axis',(-1.,0.,0.));
#22133=DIRECTION('ref_axis',(0.,0.,1.));
#44959=CARTESIAN_POINT('',(0.,0.,0.));
#44960=CARTESIAN_POINT('Origin',(4.1,-3.5,-6.06217782649107));
#44961=CARTESIAN_POINT('',(4.1,-3.5,-5.46217782649107));
#44962=CARTESIAN_POINT('Origin',(4.1,-3.5,-6.06217782649107));
#44963=CARTESIAN_POINT('',(5.7,-3.5,-5.46217782649107));
#44964=CARTESIAN_POINT('',(4.1,-3.5,-5.46217782649107));
#44965=CARTESIAN_POINT('Origin',(5.7,-3.5,-6.06217782649107));
#44966=CARTESIAN_POINT('Origin',(5.7,-3.5,-6.06217782649107));
#44967=CARTESIAN_POINT('Origin',(4.1,7.,0.));
#44968=CARTESIAN_POINT('',(4.1,7.,0.6));
#44969=CARTESIAN_POINT('Origin',(4.1,7.,0.));
#44970=CARTESIAN_POINT('',(5.7,7.,0.6));
#44971=CARTESIAN_POINT('',(4.1,7.,0.6));
#44972=CARTESIAN_POINT('Origin',(5.7,7.,0.));
#44973=CARTESIAN_POINT('Origin',(5.7,7.,0.));
#44974=CARTESIAN_POINT('Origin',(4.1,3.5,6.06217782649107));
#44975=CARTESIAN_POINT('',(4.1,3.5,6.66217782649107));
#44976=CARTESIAN_POINT('Origin',(4.1,3.5,6.06217782649107));
#44977=CARTESIAN_POINT('',(5.7,3.5,6.66217782649107));
#44978=CARTESIAN_POINT('',(4.1,3.5,6.66217782649107));
#44979=CARTESIAN_POINT('Origin',(5.7,3.5,6.06217782649107));
#44980=CARTESIAN_POINT('Origin',(5.7,3.5,6.06217782649107));
#44981=CARTESIAN_POINT('Origin',(4.1,-3.5,6.06217782649107));
#44982=CARTESIAN_POINT('',(4.1,-3.5,6.66217782649107));
#44983=CARTESIAN_POINT('Origin',(4.1,-3.5,6.06217782649107));
#44984=CARTESIAN_POINT('',(5.7,-3.5,6.66217782649107));
#44985=CARTESIAN_POINT('',(4.1,-3.5,6.66217782649107));
#44986=CARTESIAN_POINT('Origin',(5.7,-3.5,6.06217782649107));
#44987=CARTESIAN_POINT('Origin',(5.7,-3.5,6.06217782649107));
#44988=CARTESIAN_POINT('Origin',(4.1,-7.,8.57252759403147E-16));
#44989=CARTESIAN_POINT('',(4.1,-7.,0.600000000000001));
#44990=CARTESIAN_POINT('Origin',(4.1,-7.,8.57252759403147E-16));
#44991=CARTESIAN_POINT('',(5.7,-7.,0.600000000000001));
#44992=CARTESIAN_POINT('',(4.1,-7.,0.600000000000001));
#44993=CARTESIAN_POINT('Origin',(5.7,-7.,8.57252759403147E-16));
#44994=CARTESIAN_POINT('Origin',(5.7,-7.,8.32667268468867E-16));
#44995=CARTESIAN_POINT('Origin',(4.1,3.5,-6.06217782649107));
#44996=CARTESIAN_POINT('',(4.1,3.5,-5.46217782649107));
#44997=CARTESIAN_POINT('Origin',(4.1,3.5,-6.06217782649107));
#44998=CARTESIAN_POINT('',(5.7,3.5,-5.46217782649107));
#44999=CARTESIAN_POINT('',(4.1,3.5,-5.46217782649107));
#45000=CARTESIAN_POINT('Origin',(5.7,3.5,-6.06217782649107));
#45001=CARTESIAN_POINT('Origin',(5.7,3.5,-6.06217782649107));
#45002=CARTESIAN_POINT('Origin',(10.325,0.,0.));
#45003=CARTESIAN_POINT('',(9.5,-6.6,-8.08266887437253E-16));
#45004=CARTESIAN_POINT('Origin',(9.5,0.,0.));
#45005=CARTESIAN_POINT('',(11.15,-6.6,-8.08266887437253E-16));
#45006=CARTESIAN_POINT('',(10.325,-6.6,-8.08266887437253E-16));
#45007=CARTESIAN_POINT('Origin',(11.15,0.,0.));
#45008=CARTESIAN_POINT('Origin',(9.5,8.,0.));
#45009=CARTESIAN_POINT('',(9.5,-7.6,9.30731567351989E-16));
#45010=CARTESIAN_POINT('Origin',(9.5,0.,0.));
#45011=CARTESIAN_POINT('Origin',(11.15,6.6,0.));
#45012=CARTESIAN_POINT('',(11.15,-7.6,-9.30731567351989E-16));
#45013=CARTESIAN_POINT('Origin',(11.15,0.,0.));
#45014=CARTESIAN_POINT('Origin',(10.55,0.,0.));
#45015=CARTESIAN_POINT('',(15.2,-7.6,-9.30731567351989E-16));
#45016=CARTESIAN_POINT('Origin',(15.2,0.,0.));
#45017=CARTESIAN_POINT('',(10.55,-7.6,-9.30731567351989E-16));
#45018=CARTESIAN_POINT('Origin',(0.1,0.,0.));
#45019=CARTESIAN_POINT('',(0.2,-5.75,-7.04171909509728E-16));
#45020=CARTESIAN_POINT('Origin',(0.2,0.,0.));
#45021=CARTESIAN_POINT('',(-1.04083408558608E-16,-5.55,-6.79678973526781E-16));
#45022=CARTESIAN_POINT('',(0.1,-5.65,-6.91925441518255E-16));
#45023=CARTESIAN_POINT('Origin',(0.,0.,0.));
#45024=CARTESIAN_POINT('Origin',(2.15,0.,0.));
#45025=CARTESIAN_POINT('',(4.1,-5.75,-7.04171909509728E-16));
#45026=CARTESIAN_POINT('Origin',(4.1,0.,0.));
#45027=CARTESIAN_POINT('',(2.15,-5.75,-7.04171909509728E-16));
#45028=CARTESIAN_POINT('Origin',(4.1,8.3,0.));
#45029=CARTESIAN_POINT('',(4.1,-8.3,-1.0164568432923E-15));
#45030=CARTESIAN_POINT('Origin',(4.1,0.,0.));
#45031=CARTESIAN_POINT('Origin',(4.2,0.,0.));
#45032=CARTESIAN_POINT('',(4.3,-8.5,-1.04094977927525E-15));
#45033=CARTESIAN_POINT('Origin',(4.3,0.,0.));
#45034=CARTESIAN_POINT('',(4.2,-8.4,-1.02870331128378E-15));
#45035=CARTESIAN_POINT('Origin',(4.9,0.,0.));
#45036=CARTESIAN_POINT('',(5.5,-8.5,-1.04094977927525E-15));
#45037=CARTESIAN_POINT('Origin',(5.5,0.,0.));
#45038=CARTESIAN_POINT('',(4.9,-8.5,-1.04094977927525E-15));
#45039=CARTESIAN_POINT('Origin',(5.6,0.,0.));
#45040=CARTESIAN_POINT('',(5.7,-8.3,-1.0164568432923E-15));
#45041=CARTESIAN_POINT('Origin',(5.7,0.,0.));
#45042=CARTESIAN_POINT('',(5.6,-8.4,-1.02870331128378E-15));
#45043=CARTESIAN_POINT('Origin',(5.7,7.8,0.));
#45044=CARTESIAN_POINT('',(5.7,-7.8,-9.55224503334935E-16));
#45045=CARTESIAN_POINT('Origin',(5.7,0.,0.));
#45046=CARTESIAN_POINT('Origin',(5.8,0.,0.));
#45047=CARTESIAN_POINT('',(5.9,-7.6,-9.30731567351989E-16));
#45048=CARTESIAN_POINT('Origin',(5.9,0.,0.));
#45049=CARTESIAN_POINT('',(5.8,-7.7,-9.42978035343462E-16));
#45050=CARTESIAN_POINT('Origin',(10.55,0.,0.));
#45051=CARTESIAN_POINT('',(10.55,-7.6,-9.30731567351989E-16));
#45052=CARTESIAN_POINT('Origin',(15.35,0.,0.));
#45053=CARTESIAN_POINT('',(15.5,-7.3,-8.93992163377568E-16));
#45054=CARTESIAN_POINT('Origin',(15.5,0.,0.));
#45055=CARTESIAN_POINT('',(15.35,-7.45,-9.12361865364778E-16));
#45056=CARTESIAN_POINT('Origin',(15.5,3.81,0.));
#45057=CARTESIAN_POINT('',(15.5,-3.81,-4.66590430475142E-16));
#45058=CARTESIAN_POINT('Origin',(15.5,0.,0.));
#45059=CARTESIAN_POINT('Origin',(15.35,0.,0.));
#45060=CARTESIAN_POINT('',(15.2,-3.505,-4.29238703101147E-16));
#45061=CARTESIAN_POINT('',(15.35,-3.6575,-4.47914566788144E-16));
#45062=CARTESIAN_POINT('Origin',(15.2,0.,0.));
#45063=CARTESIAN_POINT('Origin',(7.75,0.,0.));
#45064=CARTESIAN_POINT('',(0.299999999999999,-3.505,-4.29238703101147E-16));
#45065=CARTESIAN_POINT('',(7.75,-3.505,-4.29238703101147E-16));
#45066=CARTESIAN_POINT('Origin',(0.3,0.,0.));
#45067=CARTESIAN_POINT('Origin',(0.15,0.,0.));
#45068=CARTESIAN_POINT('',(1.21430643318376E-16,-3.81,-4.66590430475142E-16));
#45069=CARTESIAN_POINT('',(0.15,-3.6575,-4.47914566788144E-16));
#45070=CARTESIAN_POINT('Origin',(0.,0.,0.));
#45071=CARTESIAN_POINT('Origin',(0.,5.55,0.));
#60347=UNCERTAINTY_MEASURE_WITH_UNIT(LENGTH_MEASURE(0.01),#60366,
'DISTANCE_ACCURACY_VALUE',
'Maximum model space distance between geometric entities at asserted c
onnectivities');
#60353=UNCERTAINTY_MEASURE_WITH_UNIT(LENGTH_MEASURE(0.01),#60366,
'DISTANCE_ACCURACY_VALUE',
'Maximum model space distance between geometric entities at asserted c
onnectivities');
#60359=(
GEOMETRIC_REPRESENTATION_CONTEXT(3)
GLOBAL_UNCERTAINTY_ASSIGNED_CONTEXT((#60347))
GLOBAL_UNIT_ASSIGNED_CONTEXT((#60366,#60368,#60369))
REPRESENTATION_CONTEXT('','3D')
);
#60365=(
GEOMETRIC_REPRESENTATION_CONTEXT(3)
GLOBAL_UNCERTAINTY_ASSIGNED_CONTEXT((#60353))
GLOBAL_UNIT_ASSIGNED_CONTEXT((#60366,#60368,#60369))
REPRESENTATION_CONTEXT('','3D')
);
#60366=(
LENGTH_UNIT()
NAMED_UNIT(*)
SI_UNIT(.MILLI.,.METRE.)
);
#60368=(
NAMED_UNIT(*)
PLANE_ANGLE_UNIT()
SI_UNIT($,.RADIAN.)
);
#60369=(
NAMED_UNIT(*)
SI_UNIT($,.STERADIAN.)
SOLID_ANGLE_UNIT()
);
#60375=SHAPE_DEFINITION_REPRESENTATION(#60386,#60411);
#60386=PRODUCT_DEFINITION_SHAPE('',$,#60423);
#60411=SHAPE_REPRESENTATION('',(#19163),#60359);
#60417=PRODUCT_DEFINITION_CONTEXT('part definition',#60452,'design');
#60423=PRODUCT_DEFINITION('2026-10-25-00-06-35-053','07_Oil_Flinger',#60434,
#60417);
#60434=PRODUCT_DEFINITION_FORMATION('',$,#60459);
#60452=APPLICATION_CONTEXT(
'Core Data for Automotive Mechanical Design Process');
#60453=PRODUCT_CONTEXT('part definition',#60452,'mechanical');
#60459=PRODUCT('2026-10-25-00-06-35-053','07_Oil_Flinger',$,(#60453));
#60514=COLOUR_RGB('Sky Blue',0.24,0.69,0.87);
#60515=FILL_AREA_STYLE_COLOUR('',#60514);
#60516=FILL_AREA_STYLE('',(#60515));
#60517=SURFACE_STYLE_FILL_AREA(#60516);
#60518=SURFACE_SIDE_STYLE('',(#60517));
#60519=SURFACE_STYLE_USAGE(.BOTH.,#60518);
#60520=PRESENTATION_STYLE_ASSIGNMENT((#60519));
ENDSEC;
END-ISO-10303-21;
